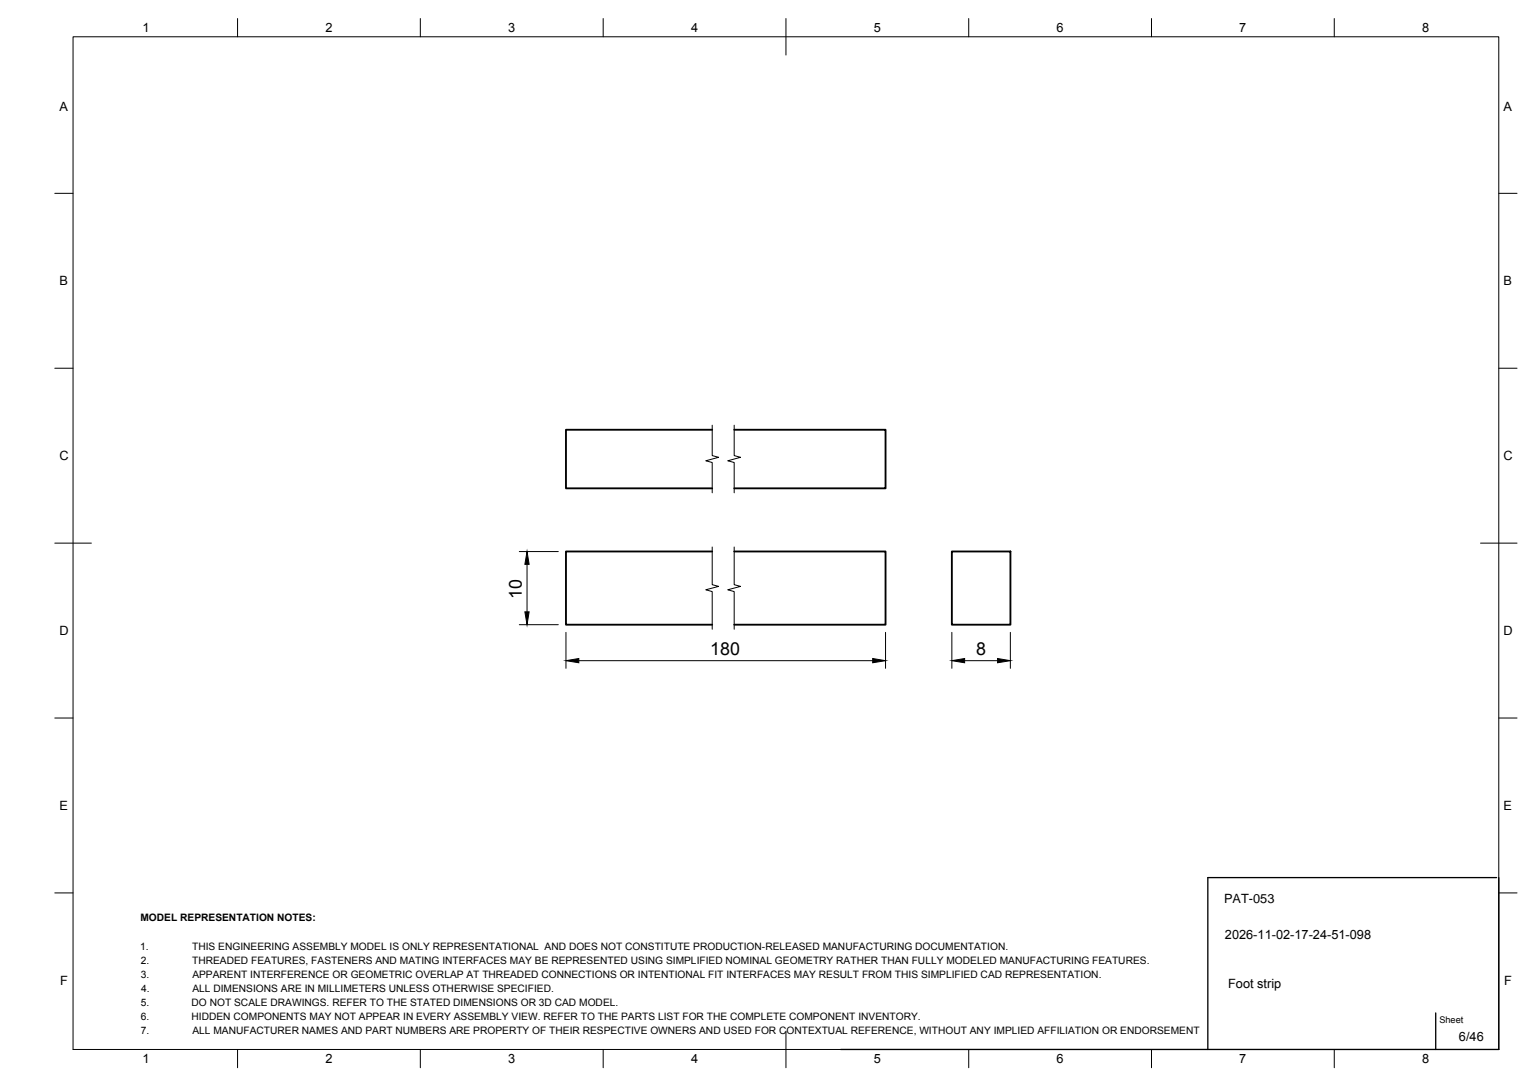
ISO-10303-21;
HEADER;
/* Generated by software containing ST-Developer
 * from STEP Tools, Inc. (www.steptools.com) 
 */

FILE_DESCRIPTION(
/* description */ ('Hand-operated arbor press'),
/* implementation_level */ '2;1');

FILE_NAME(
/* name */ 'Foot strip.step',
/* time_stamp */ '2026-10-28T03:25:25-07:00',
/* author */ (''),
/* organization */ (''),
/* preprocessor_version */ 'ST-DEVELOPER v20.2',
/* originating_system */ 'Autodesk Translation Framework v15.17.0.0',
/* authorisation */ '');

FILE_SCHEMA (('AUTOMOTIVE_DESIGN { 1 0 10303 214 3 1 1 }'));
ENDSEC;

DATA;
#10=MECHANICAL_DESIGN_GEOMETRIC_PRESENTATION_REPRESENTATION('',(#587),#32751);
#503=SHAPE_REPRESENTATION_RELATIONSHIP('SRR','None',#32932,#545);
#545=ADVANCED_BREP_SHAPE_REPRESENTATION('',(#636),#32706);
#587=STYLED_ITEM('',(#33228),#636);
#636=MANIFOLD_SOLID_BREP('Body1',#12484);
#855=PLANE('',#13039);
#856=PLANE('',#13040);
#857=PLANE('',#13041);
#858=PLANE('',#13042);
#859=PLANE('',#13043);
#860=PLANE('',#13044);
#1309=FACE_OUTER_BOUND('',#2010,.T.);
#1310=FACE_OUTER_BOUND('',#2011,.T.);
#1311=FACE_OUTER_BOUND('',#2012,.T.);
#1312=FACE_OUTER_BOUND('',#2013,.T.);
#1313=FACE_OUTER_BOUND('',#2014,.T.);
#1314=FACE_OUTER_BOUND('',#2015,.T.);
#2010=EDGE_LOOP('',(#8408,#8409,#8410,#8411));
#2011=EDGE_LOOP('',(#8412,#8413,#8414,#8415));
#2012=EDGE_LOOP('',(#8416,#8417,#8418,#8419));
#2013=EDGE_LOOP('',(#8420,#8421,#8422,#8423));
#2014=EDGE_LOOP('',(#8424,#8425,#8426,#8427));
#2015=EDGE_LOOP('',(#8428,#8429,#8430,#8431));
#2846=LINE('',#17731,#4017);
#2847=LINE('',#17733,#4018);
#2848=LINE('',#17735,#4019);
#2849=LINE('',#17736,#4020);
#2850=LINE('',#17739,#4021);
#2851=LINE('',#17741,#4022);
#2852=LINE('',#17742,#4023);
#2853=LINE('',#17745,#4024);
#2854=LINE('',#17747,#4025);
#2855=LINE('',#17748,#4026);
#2856=LINE('',#17750,#4027);
#2857=LINE('',#17751,#4028);
#4017=VECTOR('',#14259,1.);
#4018=VECTOR('',#14260,1.);
#4019=VECTOR('',#14261,1.);
#4020=VECTOR('',#14262,1.);
#4021=VECTOR('',#14265,1.);
#4022=VECTOR('',#14266,1.);
#4023=VECTOR('',#14267,1.);
#4024=VECTOR('',#14270,1.);
#4025=VECTOR('',#14271,1.);
#4026=VECTOR('',#14272,1.);
#4027=VECTOR('',#14275,1.);
#4028=VECTOR('',#14276,1.);
#5584=VERTEX_POINT('',#17729);
#5585=VERTEX_POINT('',#17730);
#5586=VERTEX_POINT('',#17732);
#5587=VERTEX_POINT('',#17734);
#5588=VERTEX_POINT('',#17738);
#5589=VERTEX_POINT('',#17740);
#5590=VERTEX_POINT('',#17744);
#5591=VERTEX_POINT('',#17746);
#6707=EDGE_CURVE('',#5584,#5585,#2846,.T.);
#6708=EDGE_CURVE('',#5585,#5586,#2847,.T.);
#6709=EDGE_CURVE('',#5587,#5586,#2848,.T.);
#6710=EDGE_CURVE('',#5584,#5587,#2849,.T.);
#6711=EDGE_CURVE('',#5588,#5584,#2850,.T.);
#6712=EDGE_CURVE('',#5589,#5587,#2851,.T.);
#6713=EDGE_CURVE('',#5588,#5589,#2852,.T.);
#6714=EDGE_CURVE('',#5590,#5588,#2853,.T.);
#6715=EDGE_CURVE('',#5591,#5589,#2854,.T.);
#6716=EDGE_CURVE('',#5590,#5591,#2855,.T.);
#6717=EDGE_CURVE('',#5585,#5590,#2856,.T.);
#6718=EDGE_CURVE('',#5586,#5591,#2857,.T.);
#8408=ORIENTED_EDGE('',*,*,#6707,.T.);
#8409=ORIENTED_EDGE('',*,*,#6708,.T.);
#8410=ORIENTED_EDGE('',*,*,#6709,.F.);
#8411=ORIENTED_EDGE('',*,*,#6710,.F.);
#8412=ORIENTED_EDGE('',*,*,#6711,.T.);
#8413=ORIENTED_EDGE('',*,*,#6710,.T.);
#8414=ORIENTED_EDGE('',*,*,#6712,.F.);
#8415=ORIENTED_EDGE('',*,*,#6713,.F.);
#8416=ORIENTED_EDGE('',*,*,#6714,.T.);
#8417=ORIENTED_EDGE('',*,*,#6713,.T.);
#8418=ORIENTED_EDGE('',*,*,#6715,.F.);
#8419=ORIENTED_EDGE('',*,*,#6716,.F.);
#8420=ORIENTED_EDGE('',*,*,#6717,.T.);
#8421=ORIENTED_EDGE('',*,*,#6716,.T.);
#8422=ORIENTED_EDGE('',*,*,#6718,.F.);
#8423=ORIENTED_EDGE('',*,*,#6708,.F.);
#8424=ORIENTED_EDGE('',*,*,#6718,.T.);
#8425=ORIENTED_EDGE('',*,*,#6715,.T.);
#8426=ORIENTED_EDGE('',*,*,#6712,.T.);
#8427=ORIENTED_EDGE('',*,*,#6709,.T.);
#8428=ORIENTED_EDGE('',*,*,#6717,.F.);
#8429=ORIENTED_EDGE('',*,*,#6707,.F.);
#8430=ORIENTED_EDGE('',*,*,#6711,.F.);
#8431=ORIENTED_EDGE('',*,*,#6714,.F.);
#11818=ADVANCED_FACE('',(#1309),#855,.T.);
#11819=ADVANCED_FACE('',(#1310),#856,.T.);
#11820=ADVANCED_FACE('',(#1311),#857,.T.);
#11821=ADVANCED_FACE('',(#1312),#858,.T.);
#11822=ADVANCED_FACE('',(#1313),#859,.T.);
#11823=ADVANCED_FACE('',(#1314),#860,.F.);
#12484=CLOSED_SHELL('',(#11818,#11819,#11820,#11821,#11822,#11823));
#13038=AXIS2_PLACEMENT_3D('',#17727,#14255,#14256);
#13039=AXIS2_PLACEMENT_3D('',#17728,#14257,#14258);
#13040=AXIS2_PLACEMENT_3D('',#17737,#14263,#14264);
#13041=AXIS2_PLACEMENT_3D('',#17743,#14268,#14269);
#13042=AXIS2_PLACEMENT_3D('',#17749,#14273,#14274);
#13043=AXIS2_PLACEMENT_3D('',#17752,#14277,#14278);
#13044=AXIS2_PLACEMENT_3D('',#17753,#14279,#14280);
#14255=DIRECTION('axis',(0.,0.,1.));
#14256=DIRECTION('refdir',(1.,0.,0.));
#14257=DIRECTION('center_axis',(0.,1.,0.));
#14258=DIRECTION('ref_axis',(-1.,0.,0.));
#14259=DIRECTION('',(-1.,0.,0.));
#14260=DIRECTION('',(0.,0.,1.));
#14261=DIRECTION('',(-1.,0.,0.));
#14262=DIRECTION('',(0.,0.,1.));
#14263=DIRECTION('center_axis',(1.,0.,0.));
#14264=DIRECTION('ref_axis',(0.,1.,0.));
#14265=DIRECTION('',(0.,1.,0.));
#14266=DIRECTION('',(0.,1.,0.));
#14267=DIRECTION('',(0.,0.,1.));
#14268=DIRECTION('center_axis',(0.,-1.,0.));
#14269=DIRECTION('ref_axis',(1.,0.,0.));
#14270=DIRECTION('',(1.,0.,0.));
#14271=DIRECTION('',(1.,0.,0.));
#14272=DIRECTION('',(0.,0.,1.));
#14273=DIRECTION('center_axis',(-1.,0.,0.));
#14274=DIRECTION('ref_axis',(0.,-1.,0.));
#14275=DIRECTION('',(0.,-1.,0.));
#14276=DIRECTION('',(0.,-1.,0.));
#14277=DIRECTION('center_axis',(0.,0.,1.));
#14278=DIRECTION('ref_axis',(1.,0.,0.));
#14279=DIRECTION('center_axis',(0.,0.,1.));
#14280=DIRECTION('ref_axis',(1.,0.,0.));
#17727=CARTESIAN_POINT('',(0.,0.,0.));
#17728=CARTESIAN_POINT('Origin',(-7.,9.,-0.8));
#17729=CARTESIAN_POINT('',(-7.,9.,-0.8));
#17730=CARTESIAN_POINT('',(-8.,9.,-0.8));
#17731=CARTESIAN_POINT('',(-7.,9.,-0.8));
#17732=CARTESIAN_POINT('',(-8.,9.,0.));
#17733=CARTESIAN_POINT('',(-8.,9.,-0.8));
#17734=CARTESIAN_POINT('',(-7.,9.,0.));
#17735=CARTESIAN_POINT('',(-7.,9.,0.));
#17736=CARTESIAN_POINT('',(-7.,9.,-0.8));
#17737=CARTESIAN_POINT('Origin',(-7.,-9.,-0.8));
#17738=CARTESIAN_POINT('',(-7.,-9.,-0.8));
#17739=CARTESIAN_POINT('',(-7.,-9.,-0.8));
#17740=CARTESIAN_POINT('',(-7.,-9.,0.));
#17741=CARTESIAN_POINT('',(-7.,-9.,0.));
#17742=CARTESIAN_POINT('',(-7.,-9.,-0.8));
#17743=CARTESIAN_POINT('Origin',(-8.,-9.,-0.8));
#17744=CARTESIAN_POINT('',(-8.,-9.,-0.8));
#17745=CARTESIAN_POINT('',(-8.,-9.,-0.8));
#17746=CARTESIAN_POINT('',(-8.,-9.,0.));
#17747=CARTESIAN_POINT('',(-8.,-9.,0.));
#17748=CARTESIAN_POINT('',(-8.,-9.,-0.8));
#17749=CARTESIAN_POINT('Origin',(-8.,9.,-0.8));
#17750=CARTESIAN_POINT('',(-8.,9.,-0.8));
#17751=CARTESIAN_POINT('',(-8.,9.,0.));
#17752=CARTESIAN_POINT('Origin',(-7.5,0.,0.));
#17753=CARTESIAN_POINT('Origin',(-7.5,0.,-0.8));
#32657=UNCERTAINTY_MEASURE_WITH_UNIT(LENGTH_MEASURE(0.001),#32752,
'DISTANCE_ACCURACY_VALUE',
'Maximum model space distance between geometric entities at asserted c
onnectivities');
#32702=UNCERTAINTY_MEASURE_WITH_UNIT(LENGTH_MEASURE(0.001),#32752,
'DISTANCE_ACCURACY_VALUE',
'Maximum model space distance between geometric entities at asserted c
onnectivities');
#32706=(
GEOMETRIC_REPRESENTATION_CONTEXT(3)
GLOBAL_UNCERTAINTY_ASSIGNED_CONTEXT((#32657))
GLOBAL_UNIT_ASSIGNED_CONTEXT((#32752,#32754,#32755))
REPRESENTATION_CONTEXT('','3D')
);
#32751=(
GEOMETRIC_REPRESENTATION_CONTEXT(3)
GLOBAL_UNCERTAINTY_ASSIGNED_CONTEXT((#32702))
GLOBAL_UNIT_ASSIGNED_CONTEXT((#32752,#32754,#32755))
REPRESENTATION_CONTEXT('','3D')
);
#32752=(
LENGTH_UNIT()
NAMED_UNIT(*)
SI_UNIT(.CENTI.,.METRE.)
);
#32754=(
NAMED_UNIT(*)
PLANE_ANGLE_UNIT()
SI_UNIT($,.RADIAN.)
);
#32755=(
NAMED_UNIT(*)
SI_UNIT($,.STERADIAN.)
SOLID_ANGLE_UNIT()
);
#32759=SHAPE_DEFINITION_REPRESENTATION(#32807,#32932);
#32807=PRODUCT_DEFINITION_SHAPE('',$,#32981);
#32932=SHAPE_REPRESENTATION('',(#13038),#32706);
#32977=PRODUCT_DEFINITION_CONTEXT('part definition',#33123,'design');
#32981=PRODUCT_DEFINITION('Foot strip','Foot strip',#33029,#32977);
#33029=PRODUCT_DEFINITION_FORMATION('',$,#33128);
#33123=APPLICATION_CONTEXT(
'Core Data for Automotive Mechanical Design Process');
#33124=PRODUCT_CONTEXT('part definition',#33123,'mechanical');
#33128=PRODUCT('Foot strip','Foot strip','Foot strip',(#33124));
#33222=COLOUR_RGB('Light Blue',0.38,0.62,0.78);
#33223=FILL_AREA_STYLE_COLOUR('',#33222);
#33224=FILL_AREA_STYLE('',(#33223));
#33225=SURFACE_STYLE_FILL_AREA(#33224);
#33226=SURFACE_SIDE_STYLE('',(#33225));
#33227=SURFACE_STYLE_USAGE(.BOTH.,#33226);
#33228=PRESENTATION_STYLE_ASSIGNMENT((#33227));
ENDSEC;
END-ISO-10303-21;
